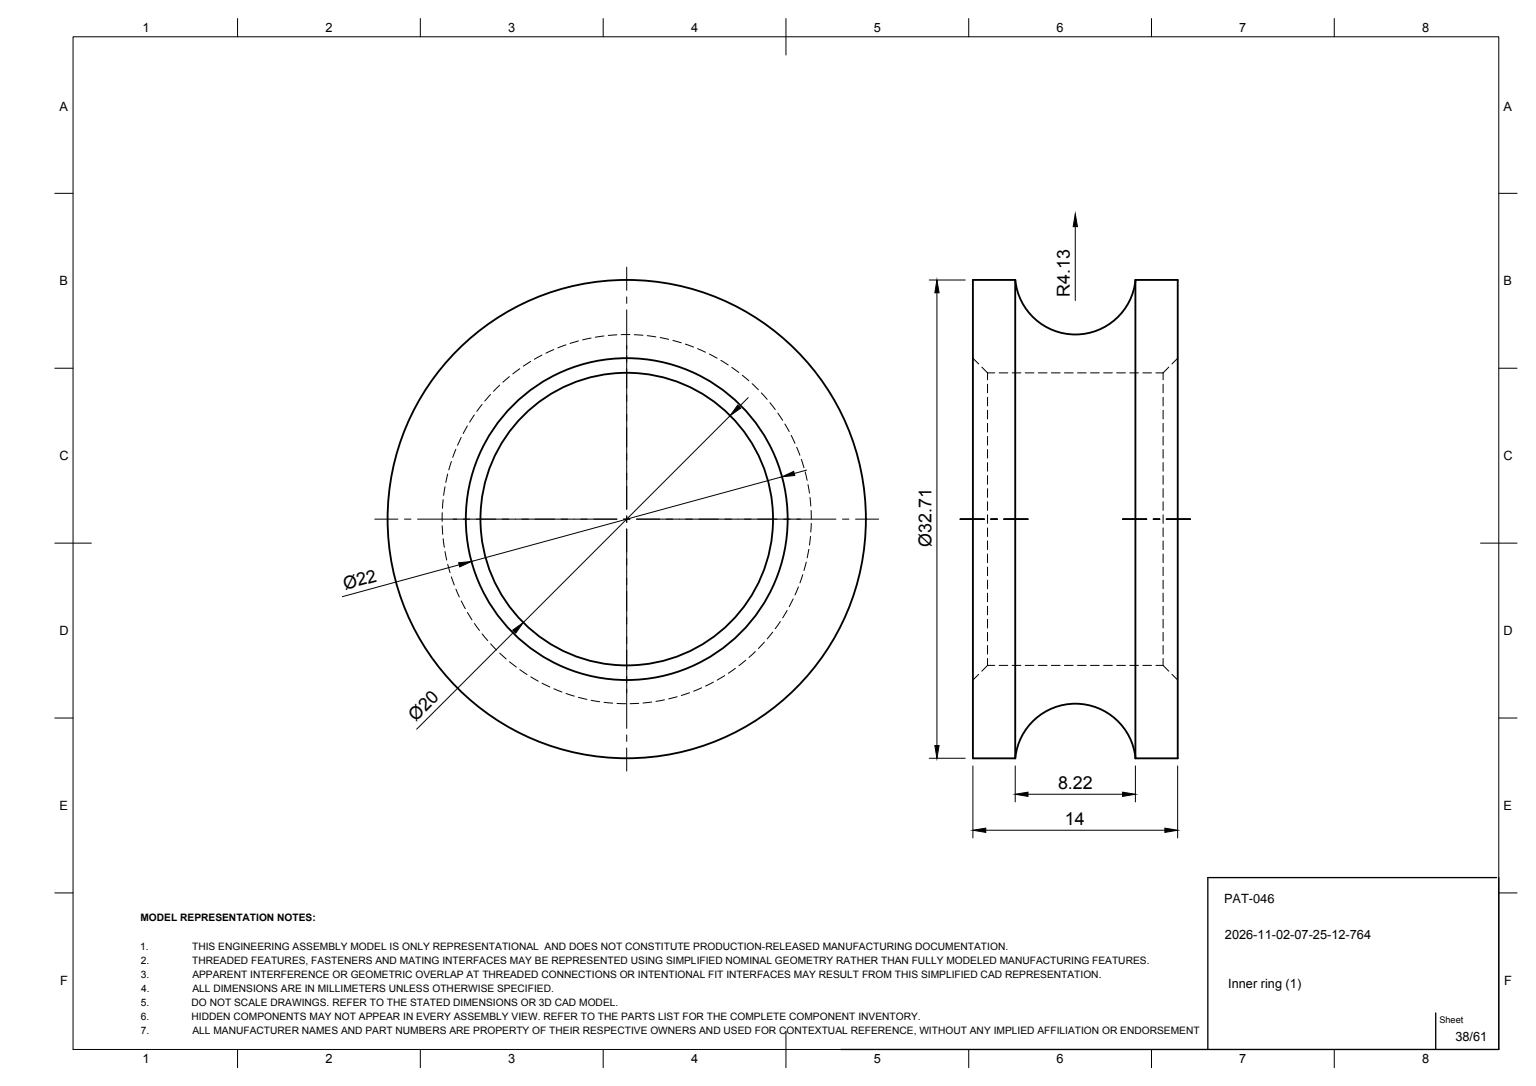
ISO-10303-21;
HEADER;
/* Generated by software containing ST-Developer
 * from STEP Tools, Inc. (www.steptools.com) 
 */

FILE_DESCRIPTION(
/* description */ ('Gear mesh backlash fixture'),
/* implementation_level */ '2;1');

FILE_NAME(
/* name */ 'Inner ring (1).step',
/* time_stamp */ '2026-10-28T03:26:00-07:00',
/* author */ (''),
/* organization */ (''),
/* preprocessor_version */ 'ST-DEVELOPER v20.2',
/* originating_system */ 'Autodesk Translation Framework v15.17.0.0',
/* authorisation */ '');

FILE_SCHEMA (('AUTOMOTIVE_DESIGN { 1 0 10303 214 3 1 1 }'));
ENDSEC;

DATA;
#10=MECHANICAL_DESIGN_GEOMETRIC_PRESENTATION_REPRESENTATION('',(#1051),#57900);
#772=CONICAL_SURFACE('',#14920,1.05,0.785398163397449);
#773=CONICAL_SURFACE('',#14927,1.05,0.785398163397449);
#782=TOROIDAL_SURFACE('',#14909,1.675,0.412776);
#944=SHAPE_REPRESENTATION_RELATIONSHIP('SRR','None',#58143,#994);
#994=ADVANCED_BREP_SHAPE_REPRESENTATION('',(#1114),#57876);
#1051=STYLED_ITEM('',(#58465),#1114);
#1114=MANIFOLD_SOLID_BREP('Body1',#13613);
#1282=FACE_BOUND('',#2953,.T.);
#1283=FACE_BOUND('',#2956,.T.);
#1532=PLANE('',#14922);
#1533=PLANE('',#14925);
#2044=FACE_OUTER_BOUND('',#2948,.T.);
#2045=FACE_OUTER_BOUND('',#2949,.T.);
#2046=FACE_OUTER_BOUND('',#2950,.T.);
#2047=FACE_OUTER_BOUND('',#2951,.T.);
#2048=FACE_OUTER_BOUND('',#2952,.T.);
#2049=FACE_OUTER_BOUND('',#2954,.T.);
#2050=FACE_OUTER_BOUND('',#2955,.T.);
#2051=FACE_OUTER_BOUND('',#2957,.T.);
#2948=EDGE_LOOP('',(#10475,#10476,#10477,#10478,#10479,#10480));
#2949=EDGE_LOOP('',(#10481,#10482,#10483,#10484,#10485));
#2950=EDGE_LOOP('',(#10486,#10487,#10488,#10489));
#2951=EDGE_LOOP('',(#10490,#10491,#10492,#10493));
#2952=EDGE_LOOP('',(#10494));
#2953=EDGE_LOOP('',(#10495));
#2954=EDGE_LOOP('',(#10496,#10497,#10498,#10499,#10500));
#2955=EDGE_LOOP('',(#10501));
#2956=EDGE_LOOP('',(#10502));
#2957=EDGE_LOOP('',(#10503,#10504,#10505,#10506));
#3863=LINE('',#21426,#4752);
#3864=LINE('',#21432,#4753);
#3865=LINE('',#21436,#4754);
#3866=LINE('',#21442,#4755);
#3867=LINE('',#21447,#4756);
#4752=VECTOR('',#17472,1.63531);
#4753=VECTOR('',#17479,1.);
#4754=VECTOR('',#17484,1.05);
#4755=VECTOR('',#17493,1.63531);
#4756=VECTOR('',#17500,1.05);
#5510=CIRCLE('',#14910,1.63531);
#5511=CIRCLE('',#14911,1.63531);
#5512=CIRCLE('',#14912,0.412776);
#5513=CIRCLE('',#14913,1.63531);
#5514=CIRCLE('',#14914,1.63531);
#5515=CIRCLE('',#14916,1.63531);
#5516=CIRCLE('',#14918,1.);
#5517=CIRCLE('',#14919,1.);
#5518=CIRCLE('',#14921,1.1);
#5519=CIRCLE('',#14924,1.63531);
#5520=CIRCLE('',#14926,1.1);
#6314=VERTEX_POINT('',#21415);
#6315=VERTEX_POINT('',#21416);
#6316=VERTEX_POINT('',#21419);
#6317=VERTEX_POINT('',#21421);
#6318=VERTEX_POINT('',#21425);
#6319=VERTEX_POINT('',#21429);
#6320=VERTEX_POINT('',#21431);
#6321=VERTEX_POINT('',#21435);
#6322=VERTEX_POINT('',#21440);
#6323=VERTEX_POINT('',#21444);
#7824=EDGE_CURVE('',#6314,#6315,#5510,.T.);
#7825=EDGE_CURVE('',#6315,#6314,#5511,.T.);
#7826=EDGE_CURVE('',#6315,#6316,#5512,.T.);
#7827=EDGE_CURVE('',#6317,#6316,#5513,.T.);
#7828=EDGE_CURVE('',#6316,#6317,#5514,.T.);
#7829=EDGE_CURVE('',#6317,#6318,#3863,.T.);
#7830=EDGE_CURVE('',#6318,#6318,#5515,.T.);
#7831=EDGE_CURVE('',#6319,#6319,#5516,.T.);
#7832=EDGE_CURVE('',#6319,#6320,#3864,.T.);
#7833=EDGE_CURVE('',#6320,#6320,#5517,.T.);
#7834=EDGE_CURVE('',#6320,#6321,#3865,.T.);
#7835=EDGE_CURVE('',#6321,#6321,#5518,.T.);
#7836=EDGE_CURVE('',#6322,#6322,#5519,.T.);
#7837=EDGE_CURVE('',#6322,#6314,#3866,.T.);
#7838=EDGE_CURVE('',#6323,#6323,#5520,.T.);
#7839=EDGE_CURVE('',#6323,#6319,#3867,.T.);
#10475=ORIENTED_EDGE('',*,*,#7824,.F.);
#10476=ORIENTED_EDGE('',*,*,#7825,.F.);
#10477=ORIENTED_EDGE('',*,*,#7826,.T.);
#10478=ORIENTED_EDGE('',*,*,#7827,.F.);
#10479=ORIENTED_EDGE('',*,*,#7828,.F.);
#10480=ORIENTED_EDGE('',*,*,#7826,.F.);
#10481=ORIENTED_EDGE('',*,*,#7827,.T.);
#10482=ORIENTED_EDGE('',*,*,#7828,.T.);
#10483=ORIENTED_EDGE('',*,*,#7829,.T.);
#10484=ORIENTED_EDGE('',*,*,#7830,.T.);
#10485=ORIENTED_EDGE('',*,*,#7829,.F.);
#10486=ORIENTED_EDGE('',*,*,#7831,.T.);
#10487=ORIENTED_EDGE('',*,*,#7832,.T.);
#10488=ORIENTED_EDGE('',*,*,#7833,.F.);
#10489=ORIENTED_EDGE('',*,*,#7832,.F.);
#10490=ORIENTED_EDGE('',*,*,#7833,.T.);
#10491=ORIENTED_EDGE('',*,*,#7834,.T.);
#10492=ORIENTED_EDGE('',*,*,#7835,.F.);
#10493=ORIENTED_EDGE('',*,*,#7834,.F.);
#10494=ORIENTED_EDGE('',*,*,#7830,.F.);
#10495=ORIENTED_EDGE('',*,*,#7835,.T.);
#10496=ORIENTED_EDGE('',*,*,#7836,.F.);
#10497=ORIENTED_EDGE('',*,*,#7837,.T.);
#10498=ORIENTED_EDGE('',*,*,#7824,.T.);
#10499=ORIENTED_EDGE('',*,*,#7825,.T.);
#10500=ORIENTED_EDGE('',*,*,#7837,.F.);
#10501=ORIENTED_EDGE('',*,*,#7836,.T.);
#10502=ORIENTED_EDGE('',*,*,#7838,.F.);
#10503=ORIENTED_EDGE('',*,*,#7838,.T.);
#10504=ORIENTED_EDGE('',*,*,#7839,.T.);
#10505=ORIENTED_EDGE('',*,*,#7831,.F.);
#10506=ORIENTED_EDGE('',*,*,#7839,.F.);
#12704=CYLINDRICAL_SURFACE('',#14915,1.63531);
#12705=CYLINDRICAL_SURFACE('',#14917,1.);
#12706=CYLINDRICAL_SURFACE('',#14923,1.63531);
#13161=ADVANCED_FACE('',(#2044),#782,.F.);
#13162=ADVANCED_FACE('',(#2045),#12704,.T.);
#13163=ADVANCED_FACE('',(#2046),#12705,.F.);
#13164=ADVANCED_FACE('',(#2047),#772,.F.);
#13165=ADVANCED_FACE('',(#2048,#1282),#1532,.T.);
#13166=ADVANCED_FACE('',(#2049),#12706,.T.);
#13167=ADVANCED_FACE('',(#2050,#1283),#1533,.T.);
#13168=ADVANCED_FACE('',(#2051),#773,.F.);
#13613=CLOSED_SHELL('',(#13161,#13162,#13163,#13164,#13165,#13166,#13167,
#13168));
#14908=AXIS2_PLACEMENT_3D('',#21413,#17456,#17457);
#14909=AXIS2_PLACEMENT_3D('',#21414,#17458,#17459);
#14910=AXIS2_PLACEMENT_3D('',#21417,#17460,#17461);
#14911=AXIS2_PLACEMENT_3D('',#21418,#17462,#17463);
#14912=AXIS2_PLACEMENT_3D('',#21420,#17464,#17465);
#14913=AXIS2_PLACEMENT_3D('',#21422,#17466,#17467);
#14914=AXIS2_PLACEMENT_3D('',#21423,#17468,#17469);
#14915=AXIS2_PLACEMENT_3D('',#21424,#17470,#17471);
#14916=AXIS2_PLACEMENT_3D('',#21427,#17473,#17474);
#14917=AXIS2_PLACEMENT_3D('',#21428,#17475,#17476);
#14918=AXIS2_PLACEMENT_3D('',#21430,#17477,#17478);
#14919=AXIS2_PLACEMENT_3D('',#21433,#17480,#17481);
#14920=AXIS2_PLACEMENT_3D('',#21434,#17482,#17483);
#14921=AXIS2_PLACEMENT_3D('',#21437,#17485,#17486);
#14922=AXIS2_PLACEMENT_3D('',#21438,#17487,#17488);
#14923=AXIS2_PLACEMENT_3D('',#21439,#17489,#17490);
#14924=AXIS2_PLACEMENT_3D('',#21441,#17491,#17492);
#14925=AXIS2_PLACEMENT_3D('',#21443,#17494,#17495);
#14926=AXIS2_PLACEMENT_3D('',#21445,#17496,#17497);
#14927=AXIS2_PLACEMENT_3D('',#21446,#17498,#17499);
#17456=DIRECTION('axis',(0.,0.,1.));
#17457=DIRECTION('refdir',(1.,0.,0.));
#17458=DIRECTION('center_axis',(0.,-1.,0.));
#17459=DIRECTION('ref_axis',(0.,0.,-1.));
#17460=DIRECTION('center_axis',(0.,-1.,0.));
#17461=DIRECTION('ref_axis',(1.,0.,0.));
#17462=DIRECTION('center_axis',(0.,-1.,0.));
#17463=DIRECTION('ref_axis',(1.,0.,0.));
#17464=DIRECTION('center_axis',(1.,0.,1.22464679914735E-16));
#17465=DIRECTION('ref_axis',(-1.22464679914735E-16,0.,1.));
#17466=DIRECTION('center_axis',(0.,1.,0.));
#17467=DIRECTION('ref_axis',(1.,0.,0.));
#17468=DIRECTION('center_axis',(0.,1.,0.));
#17469=DIRECTION('ref_axis',(1.,0.,0.));
#17470=DIRECTION('center_axis',(0.,-1.,0.));
#17471=DIRECTION('ref_axis',(1.,0.,0.));
#17472=DIRECTION('',(0.,1.,0.));
#17473=DIRECTION('center_axis',(0.,-1.,0.));
#17474=DIRECTION('ref_axis',(1.,0.,0.));
#17475=DIRECTION('center_axis',(0.,-1.,0.));
#17476=DIRECTION('ref_axis',(1.,0.,0.));
#17477=DIRECTION('center_axis',(0.,-1.,0.));
#17478=DIRECTION('ref_axis',(1.,0.,0.));
#17479=DIRECTION('',(0.,1.,0.));
#17480=DIRECTION('center_axis',(0.,-1.,0.));
#17481=DIRECTION('ref_axis',(1.,0.,0.));
#17482=DIRECTION('center_axis',(0.,1.,0.));
#17483=DIRECTION('ref_axis',(1.,0.,0.));
#17484=DIRECTION('',(-0.707106781186548,0.707106781186547,-8.65956056235494E-17));
#17485=DIRECTION('center_axis',(0.,-1.,0.));
#17486=DIRECTION('ref_axis',(1.,0.,0.));
#17487=DIRECTION('center_axis',(0.,1.,0.));
#17488=DIRECTION('ref_axis',(0.,0.,1.));
#17489=DIRECTION('center_axis',(0.,-1.,0.));
#17490=DIRECTION('ref_axis',(1.,0.,0.));
#17491=DIRECTION('center_axis',(0.,-1.,0.));
#17492=DIRECTION('ref_axis',(1.,0.,0.));
#17493=DIRECTION('',(0.,1.,0.));
#17494=DIRECTION('center_axis',(0.,-1.,0.));
#17495=DIRECTION('ref_axis',(0.,0.,-1.));
#17496=DIRECTION('center_axis',(0.,-1.,0.));
#17497=DIRECTION('ref_axis',(1.,0.,0.));
#17498=DIRECTION('center_axis',(0.,-1.,0.));
#17499=DIRECTION('ref_axis',(1.,0.,0.));
#17500=DIRECTION('',(0.707106781186548,0.707106781186547,8.65956056235494E-17));
#21413=CARTESIAN_POINT('',(0.,0.,0.));
#21414=CARTESIAN_POINT('Origin',(0.,0.,0.));
#21415=CARTESIAN_POINT('',(-1.63531,-0.410863395882378,-2.00267715711366E-16));
#21416=CARTESIAN_POINT('',(-2.00267715711366E-16,-0.410863395882378,1.63531));
#21417=CARTESIAN_POINT('Origin',(0.,-0.410863395882378,0.));
#21418=CARTESIAN_POINT('Origin',(0.,-0.410863395882378,0.));
#21419=CARTESIAN_POINT('',(-2.00267715711366E-16,0.410863395882378,1.63531));
#21420=CARTESIAN_POINT('Origin',(-2.05128338857182E-16,0.,1.675));
#21421=CARTESIAN_POINT('',(-1.63531,0.410863395882378,2.00267715711366E-16));
#21422=CARTESIAN_POINT('Origin',(0.,0.410863395882378,0.));
#21423=CARTESIAN_POINT('Origin',(0.,0.410863395882378,0.));
#21424=CARTESIAN_POINT('Origin',(0.,0.,0.));
#21425=CARTESIAN_POINT('',(-1.63531,0.7,-2.00267715711366E-16));
#21426=CARTESIAN_POINT('',(-1.63531,0.,-2.00267715711366E-16));
#21427=CARTESIAN_POINT('Origin',(0.,0.7,0.));
#21428=CARTESIAN_POINT('Origin',(0.,0.,0.));
#21429=CARTESIAN_POINT('',(-1.,-0.6,-1.22464679914735E-16));
#21430=CARTESIAN_POINT('Origin',(0.,-0.6,0.));
#21431=CARTESIAN_POINT('',(-1.,0.6,-1.22464679914735E-16));
#21432=CARTESIAN_POINT('',(-1.,0.,-1.22464679914735E-16));
#21433=CARTESIAN_POINT('Origin',(0.,0.6,0.));
#21434=CARTESIAN_POINT('Origin',(0.,0.65,0.));
#21435=CARTESIAN_POINT('',(-1.1,0.7,-1.34711147906209E-16));
#21436=CARTESIAN_POINT('',(-1.05,0.65,-1.28587913910472E-16));
#21437=CARTESIAN_POINT('Origin',(0.,0.7,0.));
#21438=CARTESIAN_POINT('Origin',(1.63531,0.7,0.));
#21439=CARTESIAN_POINT('Origin',(0.,0.,0.));
#21440=CARTESIAN_POINT('',(-1.63531,-0.7,-2.00267715711366E-16));
#21441=CARTESIAN_POINT('Origin',(0.,-0.7,0.));
#21442=CARTESIAN_POINT('',(-1.63531,0.,-2.00267715711366E-16));
#21443=CARTESIAN_POINT('Origin',(1.1,-0.7,0.));
#21444=CARTESIAN_POINT('',(-1.1,-0.7,-1.34711147906209E-16));
#21445=CARTESIAN_POINT('Origin',(0.,-0.7,0.));
#21446=CARTESIAN_POINT('Origin',(0.,-0.65,0.));
#21447=CARTESIAN_POINT('',(-1.05,-0.65,-1.28587913910472E-16));
#57817=UNCERTAINTY_MEASURE_WITH_UNIT(LENGTH_MEASURE(0.001),#57901,
'DISTANCE_ACCURACY_VALUE',
'Maximum model space distance between geometric entities at asserted c
onnectivities');
#57841=UNCERTAINTY_MEASURE_WITH_UNIT(LENGTH_MEASURE(0.001),#57901,
'DISTANCE_ACCURACY_VALUE',
'Maximum model space distance between geometric entities at asserted c
onnectivities');
#57876=(
GEOMETRIC_REPRESENTATION_CONTEXT(3)
GLOBAL_UNCERTAINTY_ASSIGNED_CONTEXT((#57817))
GLOBAL_UNIT_ASSIGNED_CONTEXT((#57901,#57903,#57904))
REPRESENTATION_CONTEXT('','3D')
);
#57900=(
GEOMETRIC_REPRESENTATION_CONTEXT(3)
GLOBAL_UNCERTAINTY_ASSIGNED_CONTEXT((#57841))
GLOBAL_UNIT_ASSIGNED_CONTEXT((#57901,#57903,#57904))
REPRESENTATION_CONTEXT('','3D')
);
#57901=(
LENGTH_UNIT()
NAMED_UNIT(*)
SI_UNIT(.CENTI.,.METRE.)
);
#57903=(
NAMED_UNIT(*)
PLANE_ANGLE_UNIT()
SI_UNIT($,.RADIAN.)
);
#57904=(
NAMED_UNIT(*)
SI_UNIT($,.STERADIAN.)
SOLID_ANGLE_UNIT()
);
#57939=SHAPE_DEFINITION_REPRESENTATION(#58005,#58143);
#58005=PRODUCT_DEFINITION_SHAPE('',$,#58202);
#58143=SHAPE_REPRESENTATION('',(#14908),#57876);
#58167=PRODUCT_DEFINITION_CONTEXT('part definition',#58343,'design');
#58202=PRODUCT_DEFINITION('Inner ring (1)','Inner ring (1)',#58260,#58167);
#58260=PRODUCT_DEFINITION_FORMATION('',$,#58379);
#58343=APPLICATION_CONTEXT(
'Core Data for Automotive Mechanical Design Process');
#58344=PRODUCT_CONTEXT('part definition',#58343,'mechanical');
#58379=PRODUCT('Inner ring (1)','Inner ring (1)','Inner ring (1)',(#58344));
#58459=COLOUR_RGB('Grey',0.48,0.52,0.57);
#58460=FILL_AREA_STYLE_COLOUR('',#58459);
#58461=FILL_AREA_STYLE('',(#58460));
#58462=SURFACE_STYLE_FILL_AREA(#58461);
#58463=SURFACE_SIDE_STYLE('',(#58462));
#58464=SURFACE_STYLE_USAGE(.BOTH.,#58463);
#58465=PRESENTATION_STYLE_ASSIGNMENT((#58464));
ENDSEC;
END-ISO-10303-21;
